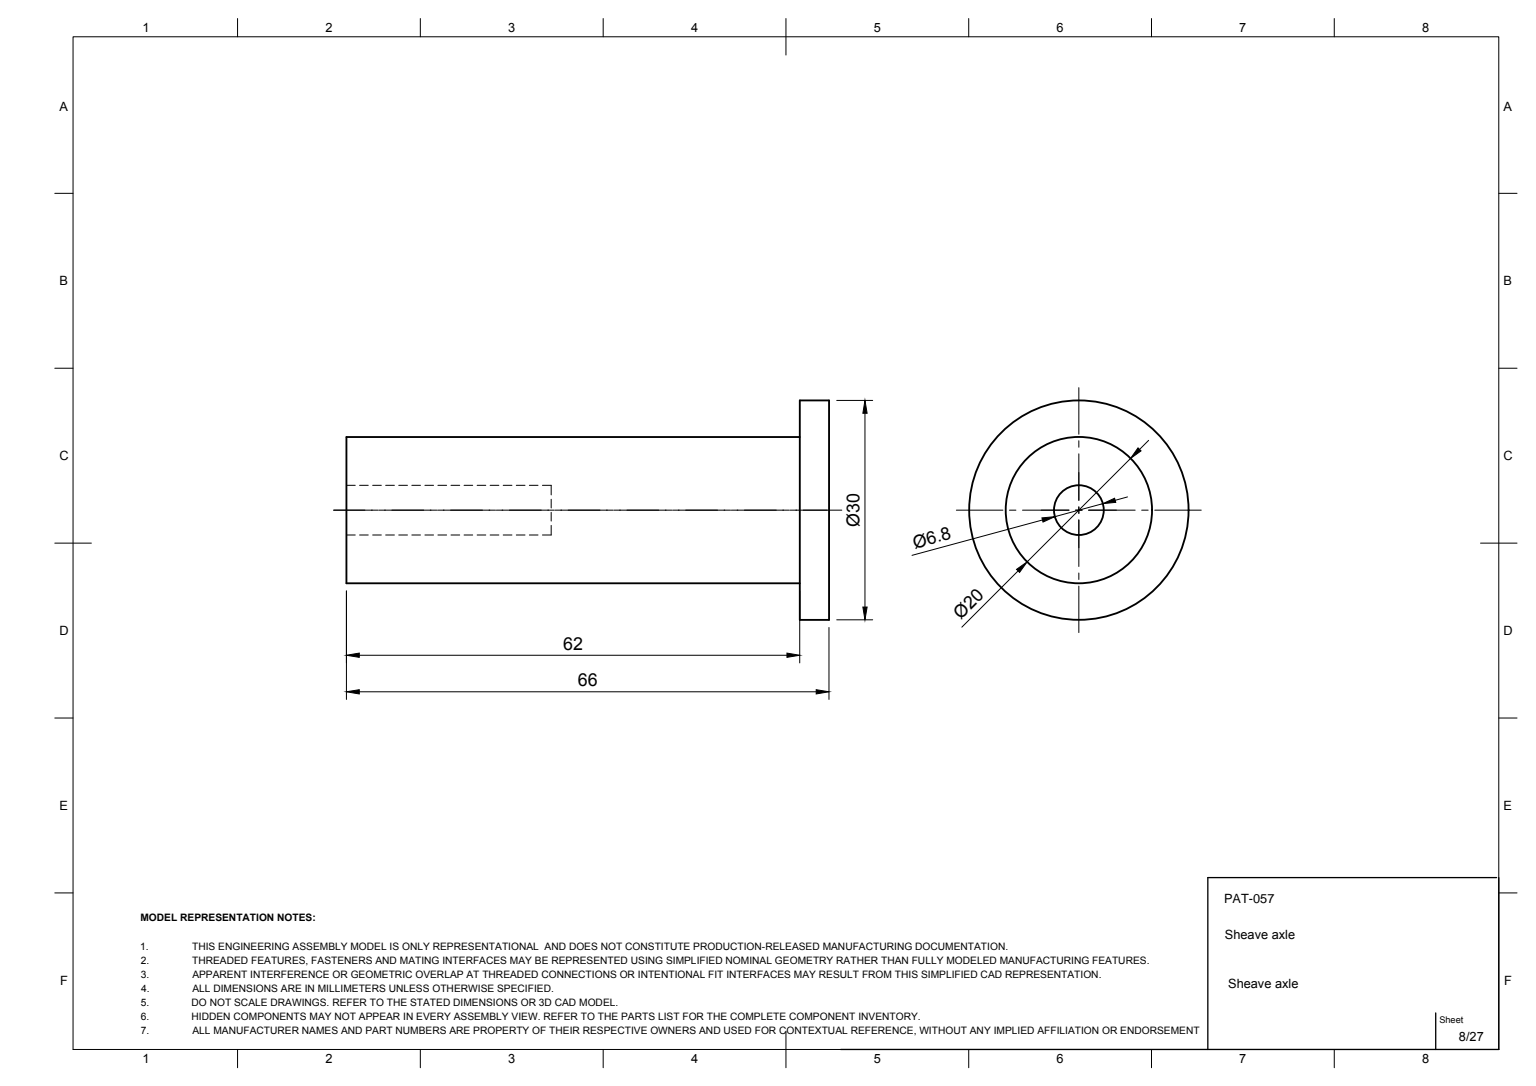
ISO-10303-21;
HEADER;
/* Generated by software containing ST-Developer
 * from STEP Tools, Inc. (www.steptools.com) 
 */

FILE_DESCRIPTION(
/* description */ ('Bearing-mounted hook block'),
/* implementation_level */ '2;1');

FILE_NAME(
/* name */ 'Sheave axle.step',
/* time_stamp */ '2026-10-28T22:30:11-07:00',
/* author */ (''),
/* organization */ (''),
/* preprocessor_version */ 'ST-DEVELOPER v20.2',
/* originating_system */ 'Autodesk Translation Framework v15.17.0.0',
/* authorisation */ '');

FILE_SCHEMA (('AUTOMOTIVE_DESIGN { 1 0 10303 214 3 1 1 }'));
ENDSEC;

DATA;
#10=MECHANICAL_DESIGN_GEOMETRIC_PRESENTATION_REPRESENTATION('',(#326),#7609);
#278=SHAPE_REPRESENTATION_RELATIONSHIP('SRR','None',#7725,#302);
#302=ADVANCED_BREP_SHAPE_REPRESENTATION('',(#358),#7585);
#326=STYLED_ITEM('',(#7931),#358);
#358=MANIFOLD_SOLID_BREP('Body1',#3922);
#442=LINE('',#6281,#672);
#443=LINE('',#6291,#673);
#444=LINE('',#6297,#674);
#672=VECTOR('',#4995,0.34);
#673=VECTOR('',#5008,1.5);
#674=VECTOR('',#5017,1.);
#862=CYLINDRICAL_SURFACE('',#4307,0.34);
#863=CYLINDRICAL_SURFACE('',#4314,1.5);
#864=CYLINDRICAL_SURFACE('',#4317,1.);
#943=FACE_BOUND('',#1300,.T.);
#944=FACE_BOUND('',#1305,.T.);
#1039=FACE_OUTER_BOUND('',#1297,.T.);
#1040=FACE_OUTER_BOUND('',#1298,.T.);
#1041=FACE_OUTER_BOUND('',#1299,.T.);
#1042=FACE_OUTER_BOUND('',#1301,.T.);
#1043=FACE_OUTER_BOUND('',#1302,.T.);
#1044=FACE_OUTER_BOUND('',#1303,.T.);
#1045=FACE_OUTER_BOUND('',#1304,.T.);
#1297=EDGE_LOOP('',(#2794,#2795,#2796,#2797));
#1298=EDGE_LOOP('',(#2798));
#1299=EDGE_LOOP('',(#2799));
#1300=EDGE_LOOP('',(#2800));
#1301=EDGE_LOOP('',(#2801,#2802,#2803,#2804));
#1302=EDGE_LOOP('',(#2805));
#1303=EDGE_LOOP('',(#2806,#2807,#2808,#2809));
#1304=EDGE_LOOP('',(#2810));
#1305=EDGE_LOOP('',(#2811));
#1597=CIRCLE('',#4308,0.34);
#1598=CIRCLE('',#4309,0.34);
#1599=CIRCLE('',#4312,1.5);
#1600=CIRCLE('',#4313,1.);
#1601=CIRCLE('',#4315,1.5);
#1602=CIRCLE('',#4318,1.);
#1846=VERTEX_POINT('',#6278);
#1847=VERTEX_POINT('',#6280);
#1848=VERTEX_POINT('',#6285);
#1849=VERTEX_POINT('',#6287);
#1850=VERTEX_POINT('',#6290);
#1851=VERTEX_POINT('',#6295);
#2207=EDGE_CURVE('',#1846,#1846,#1597,.T.);
#2208=EDGE_CURVE('',#1846,#1847,#442,.T.);
#2209=EDGE_CURVE('',#1847,#1847,#1598,.T.);
#2210=EDGE_CURVE('',#1848,#1848,#1599,.T.);
#2211=EDGE_CURVE('',#1849,#1849,#1600,.T.);
#2212=EDGE_CURVE('',#1848,#1850,#443,.T.);
#2213=EDGE_CURVE('',#1850,#1850,#1601,.T.);
#2214=EDGE_CURVE('',#1851,#1851,#1602,.T.);
#2215=EDGE_CURVE('',#1851,#1849,#444,.T.);
#2794=ORIENTED_EDGE('',*,*,#2207,.F.);
#2795=ORIENTED_EDGE('',*,*,#2208,.T.);
#2796=ORIENTED_EDGE('',*,*,#2209,.F.);
#2797=ORIENTED_EDGE('',*,*,#2208,.F.);
#2798=ORIENTED_EDGE('',*,*,#2207,.T.);
#2799=ORIENTED_EDGE('',*,*,#2210,.T.);
#2800=ORIENTED_EDGE('',*,*,#2211,.F.);
#2801=ORIENTED_EDGE('',*,*,#2210,.F.);
#2802=ORIENTED_EDGE('',*,*,#2212,.T.);
#2803=ORIENTED_EDGE('',*,*,#2213,.T.);
#2804=ORIENTED_EDGE('',*,*,#2212,.F.);
#2805=ORIENTED_EDGE('',*,*,#2213,.F.);
#2806=ORIENTED_EDGE('',*,*,#2214,.F.);
#2807=ORIENTED_EDGE('',*,*,#2215,.T.);
#2808=ORIENTED_EDGE('',*,*,#2211,.T.);
#2809=ORIENTED_EDGE('',*,*,#2215,.F.);
#2810=ORIENTED_EDGE('',*,*,#2214,.T.);
#2811=ORIENTED_EDGE('',*,*,#2209,.T.);
#3580=PLANE('',#4310);
#3581=PLANE('',#4311);
#3582=PLANE('',#4316);
#3583=PLANE('',#4319);
#3721=ADVANCED_FACE('',(#1039),#862,.F.);
#3722=ADVANCED_FACE('',(#1040),#3580,.T.);
#3723=ADVANCED_FACE('',(#1041,#943),#3581,.T.);
#3724=ADVANCED_FACE('',(#1042),#863,.T.);
#3725=ADVANCED_FACE('',(#1043),#3582,.F.);
#3726=ADVANCED_FACE('',(#1044),#864,.T.);
#3727=ADVANCED_FACE('',(#1045,#944),#3583,.T.);
#3922=CLOSED_SHELL('',(#3721,#3722,#3723,#3724,#3725,#3726,#3727));
#4306=AXIS2_PLACEMENT_3D('',#6276,#4989,#4990);
#4307=AXIS2_PLACEMENT_3D('',#6277,#4991,#4992);
#4308=AXIS2_PLACEMENT_3D('',#6279,#4993,#4994);
#4309=AXIS2_PLACEMENT_3D('',#6282,#4996,#4997);
#4310=AXIS2_PLACEMENT_3D('',#6283,#4998,#4999);
#4311=AXIS2_PLACEMENT_3D('',#6284,#5000,#5001);
#4312=AXIS2_PLACEMENT_3D('',#6286,#5002,#5003);
#4313=AXIS2_PLACEMENT_3D('',#6288,#5004,#5005);
#4314=AXIS2_PLACEMENT_3D('',#6289,#5006,#5007);
#4315=AXIS2_PLACEMENT_3D('',#6292,#5009,#5010);
#4316=AXIS2_PLACEMENT_3D('',#6293,#5011,#5012);
#4317=AXIS2_PLACEMENT_3D('',#6294,#5013,#5014);
#4318=AXIS2_PLACEMENT_3D('',#6296,#5015,#5016);
#4319=AXIS2_PLACEMENT_3D('',#6298,#5018,#5019);
#4989=DIRECTION('axis',(0.,0.,1.));
#4990=DIRECTION('refdir',(1.,0.,0.));
#4991=DIRECTION('center_axis',(0.,1.,0.));
#4992=DIRECTION('ref_axis',(1.,0.,0.));
#4993=DIRECTION('center_axis',(0.,1.,0.));
#4994=DIRECTION('ref_axis',(1.,0.,0.));
#4995=DIRECTION('',(0.,1.,0.));
#4996=DIRECTION('center_axis',(0.,-1.,0.));
#4997=DIRECTION('ref_axis',(1.,0.,0.));
#4998=DIRECTION('center_axis',(0.,1.,0.));
#4999=DIRECTION('ref_axis',(1.,0.,0.));
#5000=DIRECTION('center_axis',(0.,1.,0.));
#5001=DIRECTION('ref_axis',(1.,0.,0.));
#5002=DIRECTION('center_axis',(0.,1.,0.));
#5003=DIRECTION('ref_axis',(1.,0.,0.));
#5004=DIRECTION('center_axis',(0.,1.,0.));
#5005=DIRECTION('ref_axis',(1.,0.,0.));
#5006=DIRECTION('center_axis',(0.,1.,0.));
#5007=DIRECTION('ref_axis',(1.,0.,0.));
#5008=DIRECTION('',(0.,-1.,0.));
#5009=DIRECTION('center_axis',(0.,1.,0.));
#5010=DIRECTION('ref_axis',(1.,0.,0.));
#5011=DIRECTION('center_axis',(0.,1.,0.));
#5012=DIRECTION('ref_axis',(1.,0.,0.));
#5013=DIRECTION('center_axis',(0.,1.,0.));
#5014=DIRECTION('ref_axis',(1.,0.,0.));
#5015=DIRECTION('center_axis',(0.,1.,0.));
#5016=DIRECTION('ref_axis',(1.,0.,0.));
#5017=DIRECTION('',(0.,-1.,0.));
#5018=DIRECTION('center_axis',(0.,1.,0.));
#5019=DIRECTION('ref_axis',(1.,0.,0.));
#6276=CARTESIAN_POINT('',(0.,0.,0.));
#6277=CARTESIAN_POINT('Origin',(0.,0.3,12.));
#6278=CARTESIAN_POINT('',(-0.34,0.3,12.));
#6279=CARTESIAN_POINT('Origin',(0.,0.3,12.));
#6280=CARTESIAN_POINT('',(-0.34,3.1,12.));
#6281=CARTESIAN_POINT('',(-0.34,0.3,12.));
#6282=CARTESIAN_POINT('Origin',(0.,3.1,12.));
#6283=CARTESIAN_POINT('Origin',(0.,0.3,12.));
#6284=CARTESIAN_POINT('Origin',(0.,-3.1,12.));
#6285=CARTESIAN_POINT('',(-1.5,-3.1,12.));
#6286=CARTESIAN_POINT('Origin',(0.,-3.1,12.));
#6287=CARTESIAN_POINT('',(-1.,-3.1,12.));
#6288=CARTESIAN_POINT('Origin',(0.,-3.1,12.));
#6289=CARTESIAN_POINT('Origin',(0.,-3.5,12.));
#6290=CARTESIAN_POINT('',(-1.5,-3.5,12.));
#6291=CARTESIAN_POINT('',(-1.5,-3.5,12.));
#6292=CARTESIAN_POINT('Origin',(0.,-3.5,12.));
#6293=CARTESIAN_POINT('Origin',(0.,-3.5,12.));
#6294=CARTESIAN_POINT('Origin',(0.,-3.1,12.));
#6295=CARTESIAN_POINT('',(-1.,3.1,12.));
#6296=CARTESIAN_POINT('Origin',(0.,3.1,12.));
#6297=CARTESIAN_POINT('',(-1.,-3.1,12.));
#6298=CARTESIAN_POINT('Origin',(0.,3.1,12.));
#7555=UNCERTAINTY_MEASURE_WITH_UNIT(LENGTH_MEASURE(0.001),#7610,
'DISTANCE_ACCURACY_VALUE',
'Maximum model space distance between geometric entities at asserted c
onnectivities');
#7579=UNCERTAINTY_MEASURE_WITH_UNIT(LENGTH_MEASURE(0.001),#7610,
'DISTANCE_ACCURACY_VALUE',
'Maximum model space distance between geometric entities at asserted c
onnectivities');
#7585=(
GEOMETRIC_REPRESENTATION_CONTEXT(3)
GLOBAL_UNCERTAINTY_ASSIGNED_CONTEXT((#7555))
GLOBAL_UNIT_ASSIGNED_CONTEXT((#7610,#7612,#7613))
REPRESENTATION_CONTEXT('','3D')
);
#7609=(
GEOMETRIC_REPRESENTATION_CONTEXT(3)
GLOBAL_UNCERTAINTY_ASSIGNED_CONTEXT((#7579))
GLOBAL_UNIT_ASSIGNED_CONTEXT((#7610,#7612,#7613))
REPRESENTATION_CONTEXT('','3D')
);
#7610=(
LENGTH_UNIT()
NAMED_UNIT(*)
SI_UNIT(.CENTI.,.METRE.)
);
#7612=(
NAMED_UNIT(*)
PLANE_ANGLE_UNIT()
SI_UNIT($,.RADIAN.)
);
#7613=(
NAMED_UNIT(*)
SI_UNIT($,.STERADIAN.)
SOLID_ANGLE_UNIT()
);
#7619=SHAPE_DEFINITION_REPRESENTATION(#7648,#7725);
#7648=PRODUCT_DEFINITION_SHAPE('',$,#7755);
#7725=SHAPE_REPRESENTATION('',(#4306),#7585);
#7749=PRODUCT_DEFINITION_CONTEXT('part definition',#7838,'design');
#7755=PRODUCT_DEFINITION('Sheave axle','Sheave axle',#7784,#7749);
#7784=PRODUCT_DEFINITION_FORMATION('',$,#7845);
#7838=APPLICATION_CONTEXT(
'Core Data for Automotive Mechanical Design Process');
#7839=PRODUCT_CONTEXT('part definition',#7838,'mechanical');
#7845=PRODUCT('Sheave axle','Sheave axle','Sheave axle',(#7839));
#7925=COLOUR_RGB('Grey',0.48,0.52,0.57);
#7926=FILL_AREA_STYLE_COLOUR('',#7925);
#7927=FILL_AREA_STYLE('',(#7926));
#7928=SURFACE_STYLE_FILL_AREA(#7927);
#7929=SURFACE_SIDE_STYLE('',(#7928));
#7930=SURFACE_STYLE_USAGE(.BOTH.,#7929);
#7931=PRESENTATION_STYLE_ASSIGNMENT((#7930));
ENDSEC;
END-ISO-10303-21;
